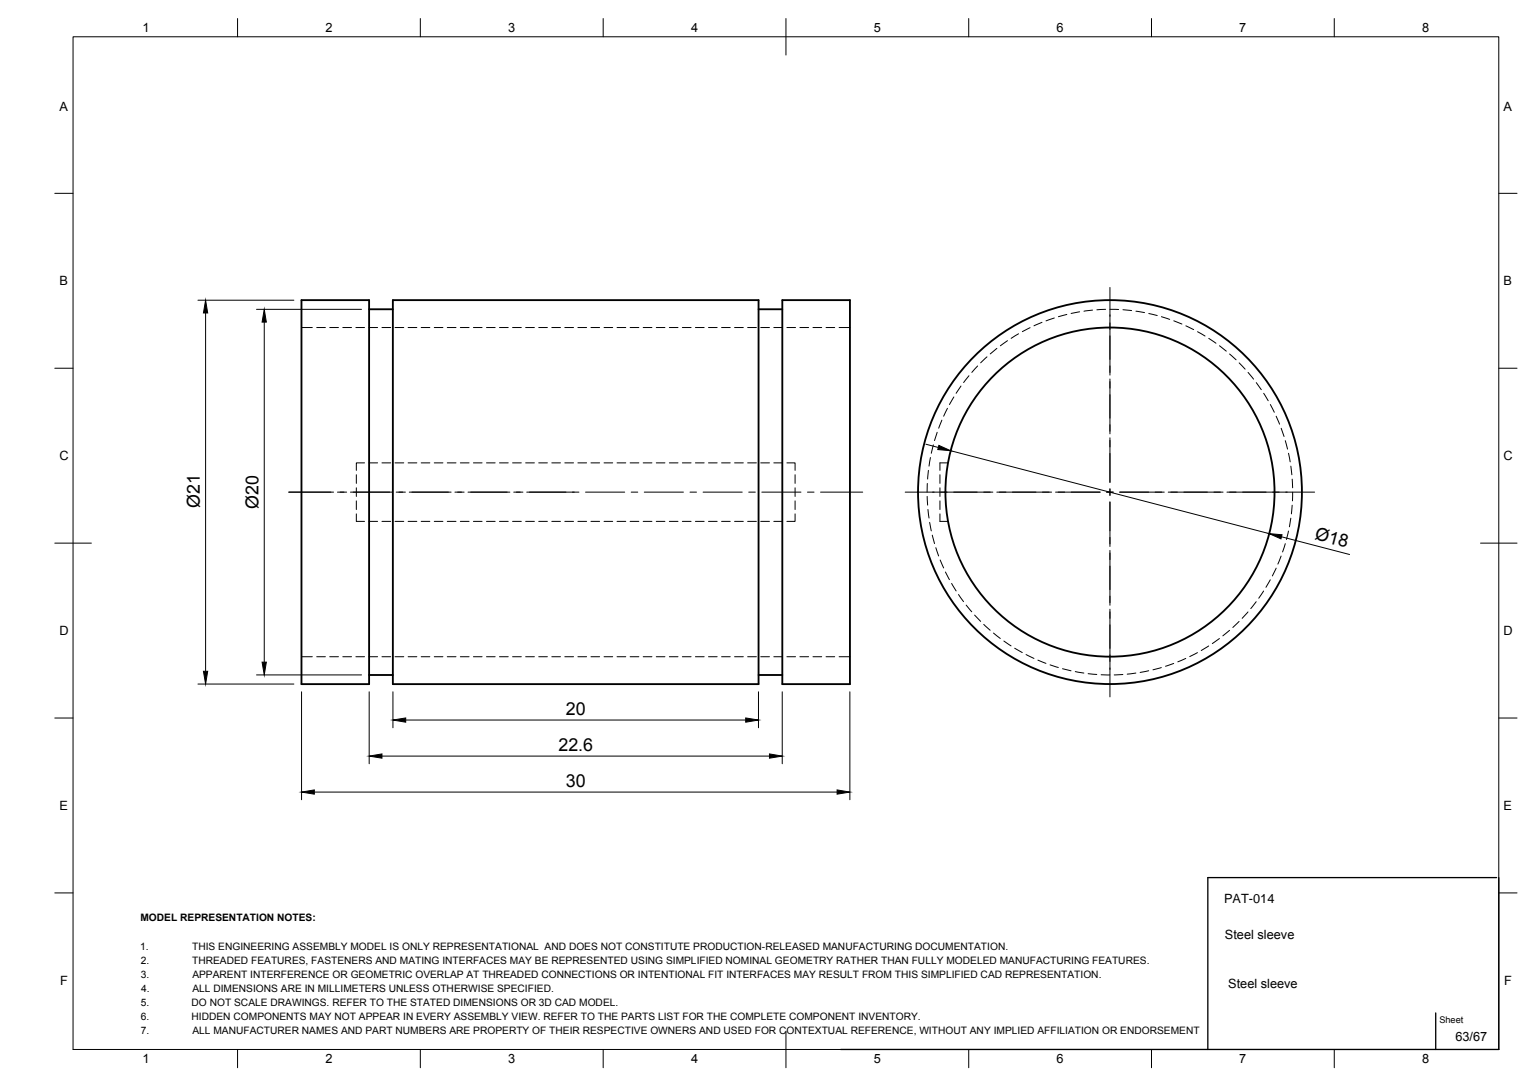
ISO-10303-21;
HEADER;
/* Generated by software containing ST-Developer
 * from STEP Tools, Inc. (www.steptools.com) 
 */

FILE_DESCRIPTION(
/* description */ ('Bin tilter linkage'),
/* implementation_level */ '2;1');

FILE_NAME(
/* name */ 'Steel sleeve.step',
/* time_stamp */ '2026-10-28T03:26:24-07:00',
/* author */ (''),
/* organization */ (''),
/* preprocessor_version */ 'ST-DEVELOPER v20.2',
/* originating_system */ 'Autodesk Translation Framework v15.17.0.0',
/* authorisation */ '');

FILE_SCHEMA (('AUTOMOTIVE_DESIGN { 1 0 10303 214 3 1 1 }'));
ENDSEC;

DATA;
#10=MECHANICAL_DESIGN_GEOMETRIC_PRESENTATION_REPRESENTATION('',(#967),#23728);
#747=SHAPE_REPRESENTATION_RELATIONSHIP('SRR','None',#24217,#853);
#853=ADVANCED_BREP_SHAPE_REPRESENTATION('',(#1079),#23717);
#967=STYLED_ITEM('',(#24779),#1079);
#1079=MANIFOLD_SOLID_BREP('Body1',#12499);
#1470=FACE_BOUND('',#3766,.T.);
#1471=FACE_BOUND('',#3769,.T.);
#1472=FACE_BOUND('',#3772,.T.);
#1473=FACE_BOUND('',#3775,.T.);
#1474=FACE_BOUND('',#3778,.T.);
#1475=FACE_BOUND('',#3781,.T.);
#1476=FACE_BOUND('',#3783,.T.);
#1848=PLANE('',#15319);
#1849=PLANE('',#15321);
#1850=PLANE('',#15322);
#1851=PLANE('',#15324);
#1852=PLANE('',#15325);
#1853=PLANE('',#15326);
#1854=PLANE('',#15331);
#1855=PLANE('',#15335);
#1856=PLANE('',#15339);
#1857=PLANE('',#15343);
#1858=PLANE('',#15347);
#2600=FACE_OUTER_BOUND('',#3760,.T.);
#2601=FACE_OUTER_BOUND('',#3761,.T.);
#2602=FACE_OUTER_BOUND('',#3762,.T.);
#2603=FACE_OUTER_BOUND('',#3763,.T.);
#2604=FACE_OUTER_BOUND('',#3764,.T.);
#2605=FACE_OUTER_BOUND('',#3765,.T.);
#2606=FACE_OUTER_BOUND('',#3767,.T.);
#2607=FACE_OUTER_BOUND('',#3768,.T.);
#2608=FACE_OUTER_BOUND('',#3770,.T.);
#2609=FACE_OUTER_BOUND('',#3771,.T.);
#2610=FACE_OUTER_BOUND('',#3773,.T.);
#2611=FACE_OUTER_BOUND('',#3774,.T.);
#2612=FACE_OUTER_BOUND('',#3776,.T.);
#2613=FACE_OUTER_BOUND('',#3777,.T.);
#2614=FACE_OUTER_BOUND('',#3779,.T.);
#2615=FACE_OUTER_BOUND('',#3780,.T.);
#2616=FACE_OUTER_BOUND('',#3782,.T.);
#3760=EDGE_LOOP('',(#11027,#11028,#11029,#11030));
#3761=EDGE_LOOP('',(#11031,#11032,#11033,#11034));
#3762=EDGE_LOOP('',(#11035,#11036,#11037,#11038));
#3763=EDGE_LOOP('',(#11039,#11040,#11041,#11042));
#3764=EDGE_LOOP('',(#11043,#11044,#11045,#11046));
#3765=EDGE_LOOP('',(#11047));
#3766=EDGE_LOOP('',(#11048));
#3767=EDGE_LOOP('',(#11049,#11050,#11051,#11052));
#3768=EDGE_LOOP('',(#11053));
#3769=EDGE_LOOP('',(#11054));
#3770=EDGE_LOOP('',(#11055,#11056,#11057,#11058));
#3771=EDGE_LOOP('',(#11059));
#3772=EDGE_LOOP('',(#11060));
#3773=EDGE_LOOP('',(#11061,#11062,#11063,#11064));
#3774=EDGE_LOOP('',(#11065));
#3775=EDGE_LOOP('',(#11066));
#3776=EDGE_LOOP('',(#11067,#11068,#11069,#11070));
#3777=EDGE_LOOP('',(#11071));
#3778=EDGE_LOOP('',(#11072));
#3779=EDGE_LOOP('',(#11073,#11074,#11075,#11076));
#3780=EDGE_LOOP('',(#11077));
#3781=EDGE_LOOP('',(#11078));
#3782=EDGE_LOOP('',(#11079,#11080,#11081,#11082));
#3783=EDGE_LOOP('',(#11083,#11084,#11085,#11086));
#4457=LINE('',#23199,#5132);
#4458=LINE('',#23201,#5133);
#4459=LINE('',#23202,#5134);
#4460=LINE('',#23205,#5135);
#4461=LINE('',#23207,#5136);
#4462=LINE('',#23208,#5137);
#4463=LINE('',#23213,#5138);
#4464=LINE('',#23214,#5139);
#4465=LINE('',#23216,#5140);
#4466=LINE('',#23217,#5141);
#4467=LINE('',#23227,#5142);
#4468=LINE('',#23234,#5143);
#4469=LINE('',#23241,#5144);
#4470=LINE('',#23248,#5145);
#4471=LINE('',#23255,#5146);
#4472=LINE('',#23260,#5147);
#5132=VECTOR('',#19372,1.);
#5133=VECTOR('',#19373,1.);
#5134=VECTOR('',#19374,1.);
#5135=VECTOR('',#19377,1.);
#5136=VECTOR('',#19378,1.);
#5137=VECTOR('',#19379,1.);
#5138=VECTOR('',#19384,1.);
#5139=VECTOR('',#19385,1.);
#5140=VECTOR('',#19388,1.);
#5141=VECTOR('',#19389,1.);
#5142=VECTOR('',#19402,1.05);
#5143=VECTOR('',#19411,1.);
#5144=VECTOR('',#19420,1.05);
#5145=VECTOR('',#19429,1.);
#5146=VECTOR('',#19438,1.05);
#5147=VECTOR('',#19445,0.9);
#5904=CIRCLE('',#15320,0.9);
#5905=CIRCLE('',#15323,0.9);
#5906=CIRCLE('',#15327,1.05);
#5907=CIRCLE('',#15328,0.9);
#5908=CIRCLE('',#15330,1.05);
#5909=CIRCLE('',#15332,1.);
#5910=CIRCLE('',#15334,1.);
#5911=CIRCLE('',#15336,1.05);
#5912=CIRCLE('',#15338,1.05);
#5913=CIRCLE('',#15340,1.);
#5914=CIRCLE('',#15342,1.);
#5915=CIRCLE('',#15344,1.05);
#5916=CIRCLE('',#15346,1.05);
#5917=CIRCLE('',#15348,0.9);
#6847=VERTEX_POINT('',#23195);
#6848=VERTEX_POINT('',#23196);
#6849=VERTEX_POINT('',#23198);
#6850=VERTEX_POINT('',#23200);
#6851=VERTEX_POINT('',#23204);
#6852=VERTEX_POINT('',#23206);
#6853=VERTEX_POINT('',#23210);
#6854=VERTEX_POINT('',#23212);
#6855=VERTEX_POINT('',#23220);
#6856=VERTEX_POINT('',#23222);
#6857=VERTEX_POINT('',#23225);
#6858=VERTEX_POINT('',#23229);
#6859=VERTEX_POINT('',#23232);
#6860=VERTEX_POINT('',#23236);
#6861=VERTEX_POINT('',#23239);
#6862=VERTEX_POINT('',#23243);
#6863=VERTEX_POINT('',#23246);
#6864=VERTEX_POINT('',#23250);
#6865=VERTEX_POINT('',#23253);
#6866=VERTEX_POINT('',#23257);
#8253=EDGE_CURVE('',#6847,#6848,#5904,.T.);
#8254=EDGE_CURVE('',#6849,#6847,#4457,.T.);
#8255=EDGE_CURVE('',#6850,#6849,#4458,.T.);
#8256=EDGE_CURVE('',#6848,#6850,#4459,.T.);
#8257=EDGE_CURVE('',#6848,#6851,#4460,.T.);
#8258=EDGE_CURVE('',#6852,#6850,#4461,.T.);
#8259=EDGE_CURVE('',#6852,#6851,#4462,.T.);
#8260=EDGE_CURVE('',#6851,#6853,#5905,.T.);
#8261=EDGE_CURVE('',#6854,#6852,#4463,.T.);
#8262=EDGE_CURVE('',#6853,#6854,#4464,.T.);
#8263=EDGE_CURVE('',#6853,#6847,#4465,.T.);
#8264=EDGE_CURVE('',#6854,#6849,#4466,.T.);
#8265=EDGE_CURVE('',#6855,#6855,#5906,.T.);
#8266=EDGE_CURVE('',#6856,#6856,#5907,.T.);
#8267=EDGE_CURVE('',#6857,#6857,#5908,.T.);
#8268=EDGE_CURVE('',#6857,#6855,#4467,.T.);
#8269=EDGE_CURVE('',#6858,#6858,#5909,.T.);
#8270=EDGE_CURVE('',#6859,#6859,#5910,.T.);
#8271=EDGE_CURVE('',#6859,#6858,#4468,.T.);
#8272=EDGE_CURVE('',#6860,#6860,#5911,.T.);
#8273=EDGE_CURVE('',#6861,#6861,#5912,.T.);
#8274=EDGE_CURVE('',#6861,#6860,#4469,.T.);
#8275=EDGE_CURVE('',#6862,#6862,#5913,.T.);
#8276=EDGE_CURVE('',#6863,#6863,#5914,.T.);
#8277=EDGE_CURVE('',#6863,#6862,#4470,.T.);
#8278=EDGE_CURVE('',#6864,#6864,#5915,.T.);
#8279=EDGE_CURVE('',#6865,#6865,#5916,.T.);
#8280=EDGE_CURVE('',#6865,#6864,#4471,.T.);
#8281=EDGE_CURVE('',#6866,#6866,#5917,.T.);
#8282=EDGE_CURVE('',#6866,#6856,#4472,.T.);
#11027=ORIENTED_EDGE('',*,*,#8253,.F.);
#11028=ORIENTED_EDGE('',*,*,#8254,.F.);
#11029=ORIENTED_EDGE('',*,*,#8255,.F.);
#11030=ORIENTED_EDGE('',*,*,#8256,.F.);
#11031=ORIENTED_EDGE('',*,*,#8257,.F.);
#11032=ORIENTED_EDGE('',*,*,#8256,.T.);
#11033=ORIENTED_EDGE('',*,*,#8258,.F.);
#11034=ORIENTED_EDGE('',*,*,#8259,.T.);
#11035=ORIENTED_EDGE('',*,*,#8260,.F.);
#11036=ORIENTED_EDGE('',*,*,#8259,.F.);
#11037=ORIENTED_EDGE('',*,*,#8261,.F.);
#11038=ORIENTED_EDGE('',*,*,#8262,.F.);
#11039=ORIENTED_EDGE('',*,*,#8263,.F.);
#11040=ORIENTED_EDGE('',*,*,#8262,.T.);
#11041=ORIENTED_EDGE('',*,*,#8264,.T.);
#11042=ORIENTED_EDGE('',*,*,#8254,.T.);
#11043=ORIENTED_EDGE('',*,*,#8264,.F.);
#11044=ORIENTED_EDGE('',*,*,#8261,.T.);
#11045=ORIENTED_EDGE('',*,*,#8258,.T.);
#11046=ORIENTED_EDGE('',*,*,#8255,.T.);
#11047=ORIENTED_EDGE('',*,*,#8265,.F.);
#11048=ORIENTED_EDGE('',*,*,#8266,.T.);
#11049=ORIENTED_EDGE('',*,*,#8267,.F.);
#11050=ORIENTED_EDGE('',*,*,#8268,.T.);
#11051=ORIENTED_EDGE('',*,*,#8265,.T.);
#11052=ORIENTED_EDGE('',*,*,#8268,.F.);
#11053=ORIENTED_EDGE('',*,*,#8267,.T.);
#11054=ORIENTED_EDGE('',*,*,#8269,.F.);
#11055=ORIENTED_EDGE('',*,*,#8270,.F.);
#11056=ORIENTED_EDGE('',*,*,#8271,.T.);
#11057=ORIENTED_EDGE('',*,*,#8269,.T.);
#11058=ORIENTED_EDGE('',*,*,#8271,.F.);
#11059=ORIENTED_EDGE('',*,*,#8272,.F.);
#11060=ORIENTED_EDGE('',*,*,#8270,.T.);
#11061=ORIENTED_EDGE('',*,*,#8273,.F.);
#11062=ORIENTED_EDGE('',*,*,#8274,.T.);
#11063=ORIENTED_EDGE('',*,*,#8272,.T.);
#11064=ORIENTED_EDGE('',*,*,#8274,.F.);
#11065=ORIENTED_EDGE('',*,*,#8273,.T.);
#11066=ORIENTED_EDGE('',*,*,#8275,.F.);
#11067=ORIENTED_EDGE('',*,*,#8276,.F.);
#11068=ORIENTED_EDGE('',*,*,#8277,.T.);
#11069=ORIENTED_EDGE('',*,*,#8275,.T.);
#11070=ORIENTED_EDGE('',*,*,#8277,.F.);
#11071=ORIENTED_EDGE('',*,*,#8278,.F.);
#11072=ORIENTED_EDGE('',*,*,#8276,.T.);
#11073=ORIENTED_EDGE('',*,*,#8279,.F.);
#11074=ORIENTED_EDGE('',*,*,#8280,.T.);
#11075=ORIENTED_EDGE('',*,*,#8278,.T.);
#11076=ORIENTED_EDGE('',*,*,#8280,.F.);
#11077=ORIENTED_EDGE('',*,*,#8279,.T.);
#11078=ORIENTED_EDGE('',*,*,#8281,.F.);
#11079=ORIENTED_EDGE('',*,*,#8281,.T.);
#11080=ORIENTED_EDGE('',*,*,#8282,.T.);
#11081=ORIENTED_EDGE('',*,*,#8266,.F.);
#11082=ORIENTED_EDGE('',*,*,#8282,.F.);
#11083=ORIENTED_EDGE('',*,*,#8260,.T.);
#11084=ORIENTED_EDGE('',*,*,#8263,.T.);
#11085=ORIENTED_EDGE('',*,*,#8253,.T.);
#11086=ORIENTED_EDGE('',*,*,#8257,.T.);
#11593=CYLINDRICAL_SURFACE('',#15329,1.05);
#11594=CYLINDRICAL_SURFACE('',#15333,1.);
#11595=CYLINDRICAL_SURFACE('',#15337,1.05);
#11596=CYLINDRICAL_SURFACE('',#15341,1.);
#11597=CYLINDRICAL_SURFACE('',#15345,1.05);
#11598=CYLINDRICAL_SURFACE('',#15349,0.9);
#12325=ADVANCED_FACE('',(#2600),#1848,.F.);
#12326=ADVANCED_FACE('',(#2601),#1849,.F.);
#12327=ADVANCED_FACE('',(#2602),#1850,.F.);
#12328=ADVANCED_FACE('',(#2603),#1851,.F.);
#12329=ADVANCED_FACE('',(#2604),#1852,.F.);
#12330=ADVANCED_FACE('',(#2605,#1470),#1853,.T.);
#12331=ADVANCED_FACE('',(#2606),#11593,.T.);
#12332=ADVANCED_FACE('',(#2607,#1471),#1854,.T.);
#12333=ADVANCED_FACE('',(#2608),#11594,.T.);
#12334=ADVANCED_FACE('',(#2609,#1472),#1855,.T.);
#12335=ADVANCED_FACE('',(#2610),#11595,.T.);
#12336=ADVANCED_FACE('',(#2611,#1473),#1856,.T.);
#12337=ADVANCED_FACE('',(#2612),#11596,.T.);
#12338=ADVANCED_FACE('',(#2613,#1474),#1857,.T.);
#12339=ADVANCED_FACE('',(#2614),#11597,.T.);
#12340=ADVANCED_FACE('',(#2615,#1475),#1858,.T.);
#12341=ADVANCED_FACE('',(#2616,#1476),#11598,.F.);
#12499=CLOSED_SHELL('',(#12325,#12326,#12327,#12328,#12329,#12330,#12331,
#12332,#12333,#12334,#12335,#12336,#12337,#12338,#12339,#12340,#12341));
#15318=AXIS2_PLACEMENT_3D('',#23193,#19366,#19367);
#15319=AXIS2_PLACEMENT_3D('',#23194,#19368,#19369);
#15320=AXIS2_PLACEMENT_3D('',#23197,#19370,#19371);
#15321=AXIS2_PLACEMENT_3D('',#23203,#19375,#19376);
#15322=AXIS2_PLACEMENT_3D('',#23209,#19380,#19381);
#15323=AXIS2_PLACEMENT_3D('',#23211,#19382,#19383);
#15324=AXIS2_PLACEMENT_3D('',#23215,#19386,#19387);
#15325=AXIS2_PLACEMENT_3D('',#23218,#19390,#19391);
#15326=AXIS2_PLACEMENT_3D('',#23219,#19392,#19393);
#15327=AXIS2_PLACEMENT_3D('',#23221,#19394,#19395);
#15328=AXIS2_PLACEMENT_3D('',#23223,#19396,#19397);
#15329=AXIS2_PLACEMENT_3D('',#23224,#19398,#19399);
#15330=AXIS2_PLACEMENT_3D('',#23226,#19400,#19401);
#15331=AXIS2_PLACEMENT_3D('',#23228,#19403,#19404);
#15332=AXIS2_PLACEMENT_3D('',#23230,#19405,#19406);
#15333=AXIS2_PLACEMENT_3D('',#23231,#19407,#19408);
#15334=AXIS2_PLACEMENT_3D('',#23233,#19409,#19410);
#15335=AXIS2_PLACEMENT_3D('',#23235,#19412,#19413);
#15336=AXIS2_PLACEMENT_3D('',#23237,#19414,#19415);
#15337=AXIS2_PLACEMENT_3D('',#23238,#19416,#19417);
#15338=AXIS2_PLACEMENT_3D('',#23240,#19418,#19419);
#15339=AXIS2_PLACEMENT_3D('',#23242,#19421,#19422);
#15340=AXIS2_PLACEMENT_3D('',#23244,#19423,#19424);
#15341=AXIS2_PLACEMENT_3D('',#23245,#19425,#19426);
#15342=AXIS2_PLACEMENT_3D('',#23247,#19427,#19428);
#15343=AXIS2_PLACEMENT_3D('',#23249,#19430,#19431);
#15344=AXIS2_PLACEMENT_3D('',#23251,#19432,#19433);
#15345=AXIS2_PLACEMENT_3D('',#23252,#19434,#19435);
#15346=AXIS2_PLACEMENT_3D('',#23254,#19436,#19437);
#15347=AXIS2_PLACEMENT_3D('',#23256,#19439,#19440);
#15348=AXIS2_PLACEMENT_3D('',#23258,#19441,#19442);
#15349=AXIS2_PLACEMENT_3D('',#23259,#19443,#19444);
#19366=DIRECTION('axis',(0.,0.,1.));
#19367=DIRECTION('refdir',(1.,0.,0.));
#19368=DIRECTION('center_axis',(0.,1.,0.));
#19369=DIRECTION('ref_axis',(0.,0.,1.));
#19370=DIRECTION('center_axis',(0.,-1.,0.));
#19371=DIRECTION('ref_axis',(1.,0.,0.));
#19372=DIRECTION('',(-1.,0.,0.));
#19373=DIRECTION('',(0.,0.,-1.));
#19374=DIRECTION('',(1.,0.,0.));
#19375=DIRECTION('center_axis',(0.,0.,1.));
#19376=DIRECTION('ref_axis',(1.,0.,0.));
#19377=DIRECTION('',(0.,-1.,0.));
#19378=DIRECTION('',(0.,1.,0.));
#19379=DIRECTION('',(-1.,0.,0.));
#19380=DIRECTION('center_axis',(0.,-1.,0.));
#19381=DIRECTION('ref_axis',(0.,0.,-1.));
#19382=DIRECTION('center_axis',(0.,1.,0.));
#19383=DIRECTION('ref_axis',(1.,0.,0.));
#19384=DIRECTION('',(0.,0.,1.));
#19385=DIRECTION('',(1.,0.,0.));
#19386=DIRECTION('center_axis',(0.,0.,-1.));
#19387=DIRECTION('ref_axis',(-1.,0.,0.));
#19388=DIRECTION('',(0.,1.,0.));
#19389=DIRECTION('',(0.,1.,0.));
#19390=DIRECTION('center_axis',(1.,0.,0.));
#19391=DIRECTION('ref_axis',(0.,0.,-1.));
#19392=DIRECTION('center_axis',(0.,1.,0.));
#19393=DIRECTION('ref_axis',(0.,0.,1.));
#19394=DIRECTION('center_axis',(0.,-1.,0.));
#19395=DIRECTION('ref_axis',(1.,0.,0.));
#19396=DIRECTION('center_axis',(0.,-1.,0.));
#19397=DIRECTION('ref_axis',(1.,0.,0.));
#19398=DIRECTION('center_axis',(0.,-1.,0.));
#19399=DIRECTION('ref_axis',(1.,0.,0.));
#19400=DIRECTION('center_axis',(0.,-1.,0.));
#19401=DIRECTION('ref_axis',(1.,0.,0.));
#19402=DIRECTION('',(0.,1.,0.));
#19403=DIRECTION('center_axis',(0.,-1.,0.));
#19404=DIRECTION('ref_axis',(0.,0.,-1.));
#19405=DIRECTION('center_axis',(0.,-1.,0.));
#19406=DIRECTION('ref_axis',(1.,0.,0.));
#19407=DIRECTION('center_axis',(0.,-1.,0.));
#19408=DIRECTION('ref_axis',(1.,0.,0.));
#19409=DIRECTION('center_axis',(0.,-1.,0.));
#19410=DIRECTION('ref_axis',(1.,0.,0.));
#19411=DIRECTION('',(0.,1.,0.));
#19412=DIRECTION('center_axis',(0.,1.,0.));
#19413=DIRECTION('ref_axis',(0.,0.,1.));
#19414=DIRECTION('center_axis',(0.,-1.,0.));
#19415=DIRECTION('ref_axis',(1.,0.,0.));
#19416=DIRECTION('center_axis',(0.,-1.,0.));
#19417=DIRECTION('ref_axis',(1.,0.,0.));
#19418=DIRECTION('center_axis',(0.,-1.,0.));
#19419=DIRECTION('ref_axis',(1.,0.,0.));
#19420=DIRECTION('',(0.,1.,0.));
#19421=DIRECTION('center_axis',(0.,-1.,0.));
#19422=DIRECTION('ref_axis',(0.,0.,-1.));
#19423=DIRECTION('center_axis',(0.,-1.,0.));
#19424=DIRECTION('ref_axis',(1.,0.,0.));
#19425=DIRECTION('center_axis',(0.,-1.,0.));
#19426=DIRECTION('ref_axis',(1.,0.,0.));
#19427=DIRECTION('center_axis',(0.,-1.,0.));
#19428=DIRECTION('ref_axis',(1.,0.,0.));
#19429=DIRECTION('',(0.,1.,0.));
#19430=DIRECTION('center_axis',(0.,1.,0.));
#19431=DIRECTION('ref_axis',(0.,0.,1.));
#19432=DIRECTION('center_axis',(0.,-1.,0.));
#19433=DIRECTION('ref_axis',(1.,0.,0.));
#19434=DIRECTION('center_axis',(0.,-1.,0.));
#19435=DIRECTION('ref_axis',(1.,0.,0.));
#19436=DIRECTION('center_axis',(0.,-1.,0.));
#19437=DIRECTION('ref_axis',(1.,0.,0.));
#19438=DIRECTION('',(0.,1.,0.));
#19439=DIRECTION('center_axis',(0.,-1.,0.));
#19440=DIRECTION('ref_axis',(0.,0.,-1.));
#19441=DIRECTION('center_axis',(0.,-1.,0.));
#19442=DIRECTION('ref_axis',(1.,0.,0.));
#19443=DIRECTION('center_axis',(0.,-1.,0.));
#19444=DIRECTION('ref_axis',(1.,0.,0.));
#19445=DIRECTION('',(0.,1.,0.));
#23193=CARTESIAN_POINT('',(0.,0.,0.));
#23194=CARTESIAN_POINT('Origin',(0.75,1.2,0.));
#23195=CARTESIAN_POINT('',(0.885663593019381,1.2,-0.16));
#23196=CARTESIAN_POINT('',(0.885663593019381,1.2,0.16));
#23197=CARTESIAN_POINT('Origin',(0.,1.2,0.));
#23198=CARTESIAN_POINT('',(0.93,1.2,-0.16));
#23199=CARTESIAN_POINT('',(0.93,1.2,-0.16));
#23200=CARTESIAN_POINT('',(0.93,1.2,0.16));
#23201=CARTESIAN_POINT('',(0.93,1.2,0.16));
#23202=CARTESIAN_POINT('',(0.57,1.2,0.16));
#23203=CARTESIAN_POINT('Origin',(0.57,0.,0.16));
#23204=CARTESIAN_POINT('',(0.885663593019381,-1.2,0.16));
#23205=CARTESIAN_POINT('',(0.885663593019381,0.,0.16));
#23206=CARTESIAN_POINT('',(0.93,-1.2,0.16));
#23207=CARTESIAN_POINT('',(0.93,0.,0.16));
#23208=CARTESIAN_POINT('',(0.57,-1.2,0.16));
#23209=CARTESIAN_POINT('Origin',(0.75,-1.2,0.));
#23210=CARTESIAN_POINT('',(0.885663593019381,-1.2,-0.16));
#23211=CARTESIAN_POINT('Origin',(0.,-1.2,0.));
#23212=CARTESIAN_POINT('',(0.93,-1.2,-0.16));
#23213=CARTESIAN_POINT('',(0.93,-1.2,0.16));
#23214=CARTESIAN_POINT('',(0.93,-1.2,-0.16));
#23215=CARTESIAN_POINT('Origin',(0.93,0.,-0.16));
#23216=CARTESIAN_POINT('',(0.885663593019381,0.,-0.16));
#23217=CARTESIAN_POINT('',(0.93,0.,-0.16));
#23218=CARTESIAN_POINT('Origin',(0.93,0.,0.16));
#23219=CARTESIAN_POINT('Origin',(1.05,1.5,0.));
#23220=CARTESIAN_POINT('',(-1.05,1.5,-1.28587913910472E-16));
#23221=CARTESIAN_POINT('Origin',(0.,1.5,0.));
#23222=CARTESIAN_POINT('',(-0.9,1.5,-1.10218211923262E-16));
#23223=CARTESIAN_POINT('Origin',(0.,1.5,0.));
#23224=CARTESIAN_POINT('Origin',(0.,1.315,0.));
#23225=CARTESIAN_POINT('',(-1.05,1.13,-1.28587913910472E-16));
#23226=CARTESIAN_POINT('Origin',(0.,1.13,0.));
#23227=CARTESIAN_POINT('',(-1.05,1.315,-1.28587913910472E-16));
#23228=CARTESIAN_POINT('Origin',(1.,1.13,0.));
#23229=CARTESIAN_POINT('',(-1.,1.13,-1.22464679914735E-16));
#23230=CARTESIAN_POINT('Origin',(0.,1.13,0.));
#23231=CARTESIAN_POINT('Origin',(0.,1.065,0.));
#23232=CARTESIAN_POINT('',(-1.,1.,-1.22464679914735E-16));
#23233=CARTESIAN_POINT('Origin',(0.,1.,0.));
#23234=CARTESIAN_POINT('',(-1.,1.065,-1.22464679914735E-16));
#23235=CARTESIAN_POINT('Origin',(1.05,1.,0.));
#23236=CARTESIAN_POINT('',(-1.05,1.,-1.28587913910472E-16));
#23237=CARTESIAN_POINT('Origin',(0.,1.,0.));
#23238=CARTESIAN_POINT('Origin',(0.,0.,0.));
#23239=CARTESIAN_POINT('',(-1.05,-1.,-1.28587913910472E-16));
#23240=CARTESIAN_POINT('Origin',(0.,-1.,0.));
#23241=CARTESIAN_POINT('',(-1.05,0.,-1.28587913910472E-16));
#23242=CARTESIAN_POINT('Origin',(1.,-1.,0.));
#23243=CARTESIAN_POINT('',(-1.,-1.,-1.22464679914735E-16));
#23244=CARTESIAN_POINT('Origin',(0.,-1.,0.));
#23245=CARTESIAN_POINT('Origin',(0.,-1.065,0.));
#23246=CARTESIAN_POINT('',(-1.,-1.13,-1.22464679914735E-16));
#23247=CARTESIAN_POINT('Origin',(0.,-1.13,0.));
#23248=CARTESIAN_POINT('',(-1.,-1.065,-1.22464679914735E-16));
#23249=CARTESIAN_POINT('Origin',(1.05,-1.13,0.));
#23250=CARTESIAN_POINT('',(-1.05,-1.13,-1.28587913910472E-16));
#23251=CARTESIAN_POINT('Origin',(0.,-1.13,0.));
#23252=CARTESIAN_POINT('Origin',(0.,-1.315,0.));
#23253=CARTESIAN_POINT('',(-1.05,-1.5,-1.28587913910472E-16));
#23254=CARTESIAN_POINT('Origin',(0.,-1.5,0.));
#23255=CARTESIAN_POINT('',(-1.05,-1.315,-1.28587913910472E-16));
#23256=CARTESIAN_POINT('Origin',(0.9,-1.5,0.));
#23257=CARTESIAN_POINT('',(-0.9,-1.5,-1.10218211923262E-16));
#23258=CARTESIAN_POINT('Origin',(0.,-1.5,0.));
#23259=CARTESIAN_POINT('Origin',(0.,0.,0.));
#23260=CARTESIAN_POINT('',(-0.9,0.,-1.10218211923262E-16));
#23600=UNCERTAINTY_MEASURE_WITH_UNIT(LENGTH_MEASURE(0.001),#23729,
'DISTANCE_ACCURACY_VALUE',
'Maximum model space distance between geometric entities at asserted c
onnectivities');
#23611=UNCERTAINTY_MEASURE_WITH_UNIT(LENGTH_MEASURE(0.001),#23729,
'DISTANCE_ACCURACY_VALUE',
'Maximum model space distance between geometric entities at asserted c
onnectivities');
#23717=(
GEOMETRIC_REPRESENTATION_CONTEXT(3)
GLOBAL_UNCERTAINTY_ASSIGNED_CONTEXT((#23600))
GLOBAL_UNIT_ASSIGNED_CONTEXT((#23729,#23731,#23732))
REPRESENTATION_CONTEXT('','3D')
);
#23728=(
GEOMETRIC_REPRESENTATION_CONTEXT(3)
GLOBAL_UNCERTAINTY_ASSIGNED_CONTEXT((#23611))
GLOBAL_UNIT_ASSIGNED_CONTEXT((#23729,#23731,#23732))
REPRESENTATION_CONTEXT('','3D')
);
#23729=(
LENGTH_UNIT()
NAMED_UNIT(*)
SI_UNIT(.CENTI.,.METRE.)
);
#23731=(
NAMED_UNIT(*)
PLANE_ANGLE_UNIT()
SI_UNIT($,.RADIAN.)
);
#23732=(
NAMED_UNIT(*)
SI_UNIT($,.STERADIAN.)
SOLID_ANGLE_UNIT()
);
#23838=SHAPE_DEFINITION_REPRESENTATION(#24076,#24217);
#24076=PRODUCT_DEFINITION_SHAPE('',$,#24334);
#24217=SHAPE_REPRESENTATION('',(#15318),#23717);
#24228=PRODUCT_DEFINITION_CONTEXT('part definition',#24578,'design');
#24334=PRODUCT_DEFINITION('Steel sleeve','Steel sleeve',#24450,#24228);
#24450=PRODUCT_DEFINITION_FORMATION('',$,#24685);
#24578=APPLICATION_CONTEXT(
'Core Data for Automotive Mechanical Design Process');
#24579=PRODUCT_CONTEXT('part definition',#24578,'mechanical');
#24685=PRODUCT('Steel sleeve','Steel sleeve','Steel sleeve',(#24579));
#24773=COLOUR_RGB('Off White',0.89,0.88,0.83);
#24774=FILL_AREA_STYLE_COLOUR('',#24773);
#24775=FILL_AREA_STYLE('',(#24774));
#24776=SURFACE_STYLE_FILL_AREA(#24775);
#24777=SURFACE_SIDE_STYLE('',(#24776));
#24778=SURFACE_STYLE_USAGE(.BOTH.,#24777);
#24779=PRESENTATION_STYLE_ASSIGNMENT((#24778));
ENDSEC;
END-ISO-10303-21;
